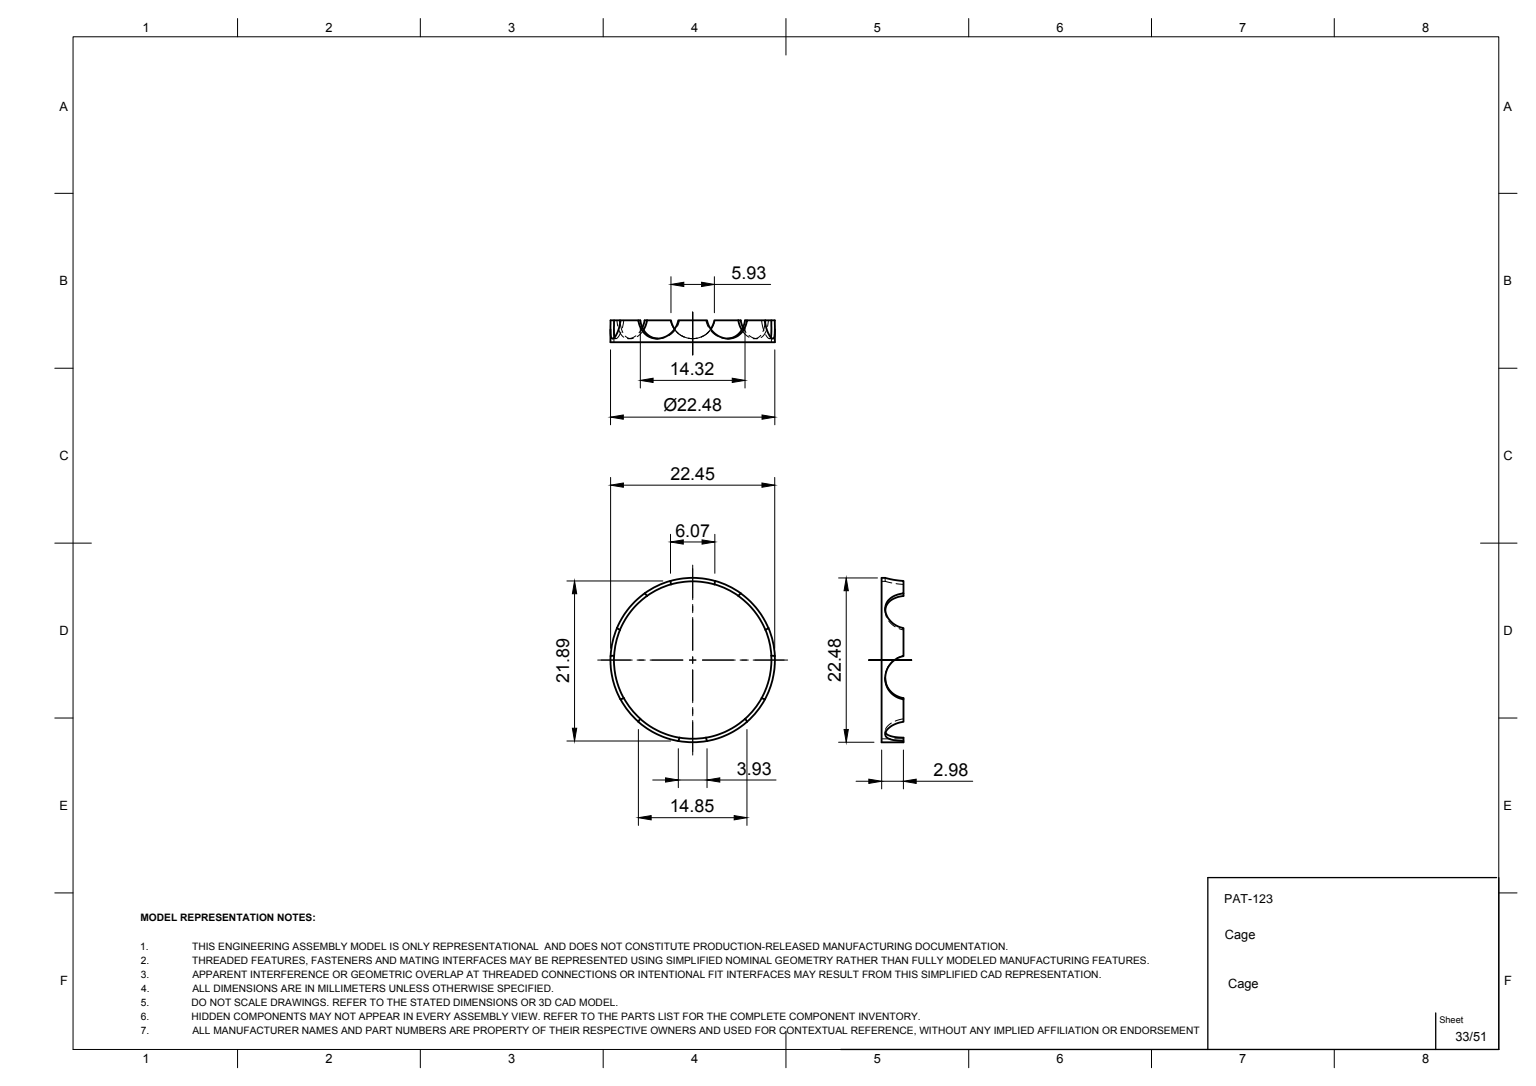
ISO-10303-21;
HEADER;
/* Generated by software containing ST-Developer
 * from STEP Tools, Inc. (www.steptools.com) 
 */

FILE_DESCRIPTION(
/* description */ ('Worm-less right-angle friction wheel drive'),
/* implementation_level */ '2;1');

FILE_NAME(
/* name */ 'Cage.step',
/* time_stamp */ '2026-10-28T03:22:36-07:00',
/* author */ (''),
/* organization */ (''),
/* preprocessor_version */ 'ST-DEVELOPER v20.2',
/* originating_system */ 'Autodesk Translation Framework v15.17.0.0',
/* authorisation */ '');

FILE_SCHEMA (('AUTOMOTIVE_DESIGN { 1 0 10303 214 3 1 1 }'));
ENDSEC;

DATA;
#10=MECHANICAL_DESIGN_GEOMETRIC_PRESENTATION_REPRESENTATION('',(#644),#17046);
#442=SPHERICAL_SURFACE('',#9318,0.309556);
#443=SPHERICAL_SURFACE('',#9334,0.309556);
#444=SPHERICAL_SURFACE('',#9339,0.309556);
#445=SPHERICAL_SURFACE('',#9345,0.309556);
#446=SPHERICAL_SURFACE('',#9350,0.309556);
#447=SPHERICAL_SURFACE('',#9355,0.309556);
#448=SPHERICAL_SURFACE('',#9363,0.309556);
#483=B_SPLINE_CURVE_WITH_KNOTS('',3,(#15498,#15499,#15500,#15501,#15502,
#15503,#15504,#15505,#15506,#15507,#15508,#15509,#15510,#15511,#15512,#15513,
#15514,#15515,#15516,#15517,#15518,#15519),.UNSPECIFIED.,.F.,.F.,(4,2,2,
2,2,2,2,2,2,2,4),(0.0591825211272536,0.157966726598481,0.236950089897721,
0.315933453196962,0.391576304923761,0.46721915665056,0.54286200837736,0.618504860104159,
0.697488223403399,0.77647158670264,0.875255792173867),.UNSPECIFIED.);
#484=B_SPLINE_CURVE_WITH_KNOTS('',3,(#15523,#15524,#15525,#15526,#15527,
#15528,#15529,#15530,#15531,#15532,#15533,#15534,#15535,#15536,#15537,#15538,
#15539,#15540,#15541,#15542,#15543,#15544),.UNSPECIFIED.,.F.,.F.,(4,2,2,
2,2,2,2,2,2,2,4),(0.0581119756758434,0.106553146291161,0.213106292582322,
0.30849933801665,0.386091982889075,0.4636846277615,0.541277272633925,0.61886991750635,
0.714262962940678,0.820816109231839,0.869257279847157),.UNSPECIFIED.);
#485=B_SPLINE_CURVE_WITH_KNOTS('',3,(#15550,#15551,#15552,#15553,#15554,
#15555,#15556,#15557,#15558,#15559,#15560,#15561,#15562,#15563,#15564,#15565,
#15566,#15567,#15568,#15569,#15570,#15571),.UNSPECIFIED.,.F.,.F.,(4,2,2,
2,2,2,2,2,2,2,4),(0.0581119756758434,0.106553146291161,0.213106292582322,
0.30849933801665,0.386091982889075,0.4636846277615,0.541277272633925,0.61886991750635,
0.714262962940679,0.820816109231839,0.869257279847157),.UNSPECIFIED.);
#486=B_SPLINE_CURVE_WITH_KNOTS('',3,(#15575,#15576,#15577,#15578,#15579,
#15580,#15581,#15582,#15583,#15584,#15585,#15586,#15587,#15588,#15589,#15590,
#15591,#15592,#15593,#15594,#15595,#15596),.UNSPECIFIED.,.F.,.F.,(4,2,2,
2,2,2,2,2,2,2,4),(0.0581119756758433,0.106553146291161,0.213106292582322,
0.308499338016649,0.386091982889075,0.4636846277615,0.541277272633925,0.61886991750635,
0.714262962940678,0.820816109231839,0.869257279847157),.UNSPECIFIED.);
#487=B_SPLINE_CURVE_WITH_KNOTS('',3,(#15605,#15606,#15607,#15608,#15609,
#15610,#15611,#15612,#15613,#15614,#15615,#15616,#15617,#15618,#15619,#15620,
#15621,#15622,#15623,#15624,#15625,#15626),.UNSPECIFIED.,.F.,.F.,(4,2,2,
2,2,2,2,2,2,2,4),(0.0581119756758433,0.106553146291161,0.213106292582322,
0.30849933801665,0.386091982889075,0.4636846277615,0.541277272633925,0.61886991750635,
0.714262962940678,0.820816109231839,0.869257279847157),.UNSPECIFIED.);
#488=B_SPLINE_CURVE_WITH_KNOTS('',3,(#15630,#15631,#15632,#15633,#15634,
#15635,#15636,#15637,#15638,#15639,#15640,#15641,#15642,#15643,#15644,#15645,
#15646,#15647,#15648,#15649,#15650,#15651),.UNSPECIFIED.,.F.,.F.,(4,2,2,
2,2,2,2,2,2,2,4),(0.0581119756758434,0.106553146291161,0.213106292582322,
0.30849933801665,0.386091982889075,0.4636846277615,0.541277272633925,0.61886991750635,
0.714262962940678,0.820816109231839,0.869257279847157),.UNSPECIFIED.);
#489=B_SPLINE_CURVE_WITH_KNOTS('',3,(#15655,#15656,#15657,#15658,#15659,
#15660,#15661,#15662,#15663,#15664,#15665,#15666,#15667,#15668,#15669,#15670,
#15671,#15672,#15673,#15674,#15675,#15676),.UNSPECIFIED.,.F.,.F.,(4,2,2,
2,2,2,2,2,2,2,4),(0.0581119756758434,0.106553146291161,0.213106292582322,
0.30849933801665,0.386091982889075,0.4636846277615,0.541277272633925,0.61886991750635,
0.714262962940678,0.820816109231839,0.869257279847157),.UNSPECIFIED.);
#490=B_SPLINE_CURVE_WITH_KNOTS('',3,(#15680,#15681,#15682,#15683,#15684,
#15685,#15686,#15687,#15688,#15689,#15690,#15691,#15692,#15693,#15694,#15695,
#15696,#15697,#15698,#15699,#15700,#15701),.UNSPECIFIED.,.F.,.F.,(4,2,2,
2,2,2,2,2,2,2,4),(0.0581119756758433,0.106553146291161,0.213106292582322,
0.30849933801665,0.386091982889075,0.4636846277615,0.541277272633925,0.61886991750635,
0.714262962940678,0.820816109231839,0.869257279847157),.UNSPECIFIED.);
#491=B_SPLINE_CURVE_WITH_KNOTS('',3,(#15709,#15710,#15711,#15712,#15713,
#15714,#15715,#15716,#15717,#15718,#15719,#15720,#15721,#15722,#15723,#15724,
#15725,#15726,#15727,#15728,#15729,#15730),.UNSPECIFIED.,.F.,.F.,(4,2,2,
2,2,2,2,2,2,2,4),(0.0591825211272536,0.157966726598481,0.236950089897721,
0.315933453196962,0.391576304923761,0.467219156650561,0.54286200837736,
0.618504860104159,0.697488223403399,0.77647158670264,0.875255792173867),
 .UNSPECIFIED.);
#492=B_SPLINE_CURVE_WITH_KNOTS('',3,(#15738,#15739,#15740,#15741,#15742,
#15743,#15744,#15745,#15746,#15747,#15748,#15749,#15750,#15751,#15752,#15753,
#15754,#15755,#15756,#15757,#15758,#15759),.UNSPECIFIED.,.F.,.F.,(4,2,2,
2,2,2,2,2,2,2,4),(0.0591825211272536,0.157966726598481,0.236950089897722,
0.315933453196962,0.391576304923761,0.467219156650561,0.54286200837736,
0.618504860104159,0.697488223403399,0.77647158670264,0.875255792173867),
 .UNSPECIFIED.);
#493=B_SPLINE_CURVE_WITH_KNOTS('',3,(#15769,#15770,#15771,#15772,#15773,
#15774,#15775,#15776,#15777,#15778,#15779,#15780,#15781,#15782,#15783,#15784,
#15785,#15786,#15787,#15788,#15789,#15790),.UNSPECIFIED.,.F.,.F.,(4,2,2,
2,2,2,2,2,2,2,4),(0.0591825211272536,0.157966726598481,0.236950089897721,
0.315933453196962,0.391576304923761,0.46721915665056,0.54286200837736,0.618504860104159,
0.697488223403399,0.77647158670264,0.875255792173867),.UNSPECIFIED.);
#494=B_SPLINE_CURVE_WITH_KNOTS('',3,(#15798,#15799,#15800,#15801,#15802,
#15803,#15804,#15805,#15806,#15807,#15808,#15809,#15810,#15811,#15812,#15813,
#15814,#15815,#15816,#15817,#15818,#15819),.UNSPECIFIED.,.F.,.F.,(4,2,2,
2,2,2,2,2,2,2,4),(0.0591825211272536,0.157966726598481,0.236950089897721,
0.315933453196962,0.391576304923761,0.46721915665056,0.542862008377359,
0.618504860104159,0.697488223403399,0.776471586702639,0.875255792173867),
 .UNSPECIFIED.);
#495=B_SPLINE_CURVE_WITH_KNOTS('',3,(#15827,#15828,#15829,#15830,#15831,
#15832,#15833,#15834,#15835,#15836,#15837,#15838,#15839,#15840,#15841,#15842,
#15843,#15844,#15845,#15846,#15847,#15848),.UNSPECIFIED.,.F.,.F.,(4,2,2,
2,2,2,2,2,2,2,4),(0.0591825211272536,0.157966726598481,0.236950089897721,
0.315933453196962,0.391576304923761,0.46721915665056,0.54286200837736,0.618504860104159,
0.697488223403399,0.77647158670264,0.875255792173867),.UNSPECIFIED.);
#496=B_SPLINE_CURVE_WITH_KNOTS('',3,(#15857,#15858,#15859,#15860,#15861,
#15862,#15863,#15864,#15865,#15866,#15867,#15868,#15869,#15870,#15871,#15872,
#15873,#15874,#15875,#15876,#15877,#15878),.UNSPECIFIED.,.F.,.F.,(4,2,2,
2,2,2,2,2,2,2,4),(0.0591825211272536,0.157966726598481,0.236950089897721,
0.315933453196962,0.391576304923761,0.46721915665056,0.542862008377359,
0.618504860104159,0.697488223403399,0.776471586702639,0.875255792173867),
 .UNSPECIFIED.);
#544=SHAPE_REPRESENTATION_RELATIONSHIP('SRR','None',#17288,#591);
#591=ADVANCED_BREP_SHAPE_REPRESENTATION('',(#697),#17024);
#644=STYLED_ITEM('',(#17591),#697);
#697=MANIFOLD_SOLID_BREP('Continuous crown cage',#8200);
#910=FACE_BOUND('',#2159,.T.);
#1083=PLANE('',#9331);
#1084=PLANE('',#9336);
#1085=PLANE('',#9341);
#1086=PLANE('',#9347);
#1087=PLANE('',#9352);
#1088=PLANE('',#9361);
#1089=PLANE('',#9365);
#1090=PLANE('',#9366);
#1482=FACE_OUTER_BOUND('',#2143,.T.);
#1483=FACE_OUTER_BOUND('',#2144,.T.);
#1484=FACE_OUTER_BOUND('',#2145,.T.);
#1485=FACE_OUTER_BOUND('',#2146,.T.);
#1486=FACE_OUTER_BOUND('',#2147,.T.);
#1487=FACE_OUTER_BOUND('',#2148,.T.);
#1488=FACE_OUTER_BOUND('',#2149,.T.);
#1489=FACE_OUTER_BOUND('',#2150,.T.);
#1490=FACE_OUTER_BOUND('',#2151,.T.);
#1491=FACE_OUTER_BOUND('',#2152,.T.);
#1492=FACE_OUTER_BOUND('',#2153,.T.);
#1493=FACE_OUTER_BOUND('',#2154,.T.);
#1494=FACE_OUTER_BOUND('',#2155,.T.);
#1495=FACE_OUTER_BOUND('',#2156,.T.);
#1496=FACE_OUTER_BOUND('',#2157,.T.);
#1497=FACE_OUTER_BOUND('',#2158,.T.);
#1498=FACE_OUTER_BOUND('',#2160,.T.);
#2143=EDGE_LOOP('',(#6744,#6745,#6746,#6747));
#2144=EDGE_LOOP('',(#6748,#6749,#6750,#6751,#6752,#6753,#6754,#6755,#6756,
#6757,#6758,#6759,#6760,#6761,#6762,#6763,#6764,#6765));
#2145=EDGE_LOOP('',(#6766,#6767,#6768,#6769));
#2146=EDGE_LOOP('',(#6770,#6771,#6772,#6773));
#2147=EDGE_LOOP('',(#6774,#6775,#6776,#6777));
#2148=EDGE_LOOP('',(#6778,#6779,#6780,#6781));
#2149=EDGE_LOOP('',(#6782,#6783,#6784,#6785,#6786,#6787));
#2150=EDGE_LOOP('',(#6788,#6789,#6790,#6791));
#2151=EDGE_LOOP('',(#6792,#6793,#6794,#6795));
#2152=EDGE_LOOP('',(#6796,#6797,#6798,#6799));
#2153=EDGE_LOOP('',(#6800,#6801,#6802,#6803));
#2154=EDGE_LOOP('',(#6804,#6805,#6806,#6807));
#2155=EDGE_LOOP('',(#6808,#6809,#6810,#6811,#6812,#6813,#6814,#6815,#6816,
#6817,#6818,#6819,#6820,#6821,#6822,#6823,#6824,#6825));
#2156=EDGE_LOOP('',(#6826,#6827,#6828,#6829));
#2157=EDGE_LOOP('',(#6830,#6831,#6832,#6833));
#2158=EDGE_LOOP('',(#6834));
#2159=EDGE_LOOP('',(#6835));
#2160=EDGE_LOOP('',(#6836,#6837,#6838,#6839));
#2707=LINE('',#15600,#3247);
#2708=LINE('',#15853,#3248);
#3247=VECTOR('',#11269,1.123812);
#3248=VECTOR('',#11338,1.076188);
#3730=CIRCLE('',#9319,0.303778037777585);
#3731=CIRCLE('',#9320,0.303778037777585);
#3732=CIRCLE('',#9322,1.123812);
#3733=CIRCLE('',#9323,1.123812);
#3734=CIRCLE('',#9324,1.123812);
#3735=CIRCLE('',#9325,1.123812);
#3736=CIRCLE('',#9326,1.123812);
#3737=CIRCLE('',#9327,1.123812);
#3738=CIRCLE('',#9328,1.123812);
#3739=CIRCLE('',#9329,1.123812);
#3740=CIRCLE('',#9330,1.123812);
#3741=CIRCLE('',#9332,1.076188);
#3742=CIRCLE('',#9333,0.303778037777585);
#3743=CIRCLE('',#9335,0.303778037777585);
#3744=CIRCLE('',#9337,1.076188);
#3745=CIRCLE('',#9338,0.303778037777585);
#3746=CIRCLE('',#9340,0.303778037777585);
#3747=CIRCLE('',#9342,1.076188);
#3748=CIRCLE('',#9343,1.076188);
#3749=CIRCLE('',#9344,0.303778037777585);
#3750=CIRCLE('',#9346,0.303778037777585);
#3751=CIRCLE('',#9348,1.076188);
#3752=CIRCLE('',#9349,0.303778037777585);
#3753=CIRCLE('',#9351,0.303778037777585);
#3754=CIRCLE('',#9353,1.076188);
#3755=CIRCLE('',#9354,0.303778037777585);
#3756=CIRCLE('',#9356,0.303778037777585);
#3757=CIRCLE('',#9358,1.076188);
#3758=CIRCLE('',#9359,1.076188);
#3759=CIRCLE('',#9360,1.076188);
#3760=CIRCLE('',#9362,0.303778037777585);
#3761=CIRCLE('',#9364,0.303778037777585);
#4279=VERTEX_POINT('',#15496);
#4280=VERTEX_POINT('',#15497);
#4281=VERTEX_POINT('',#15520);
#4282=VERTEX_POINT('',#15522);
#4283=VERTEX_POINT('',#15547);
#4284=VERTEX_POINT('',#15549);
#4285=VERTEX_POINT('',#15572);
#4286=VERTEX_POINT('',#15574);
#4287=VERTEX_POINT('',#15597);
#4288=VERTEX_POINT('',#15599);
#4289=VERTEX_POINT('',#15602);
#4290=VERTEX_POINT('',#15604);
#4291=VERTEX_POINT('',#15627);
#4292=VERTEX_POINT('',#15629);
#4293=VERTEX_POINT('',#15652);
#4294=VERTEX_POINT('',#15654);
#4295=VERTEX_POINT('',#15677);
#4296=VERTEX_POINT('',#15679);
#4297=VERTEX_POINT('',#15704);
#4298=VERTEX_POINT('',#15708);
#4299=VERTEX_POINT('',#15733);
#4300=VERTEX_POINT('',#15737);
#4301=VERTEX_POINT('',#15762);
#4302=VERTEX_POINT('',#15764);
#4303=VERTEX_POINT('',#15768);
#4304=VERTEX_POINT('',#15793);
#4305=VERTEX_POINT('',#15797);
#4306=VERTEX_POINT('',#15822);
#4307=VERTEX_POINT('',#15826);
#4308=VERTEX_POINT('',#15851);
#4309=VERTEX_POINT('',#15854);
#4310=VERTEX_POINT('',#15856);
#5141=EDGE_CURVE('',#4279,#4280,#483,.T.);
#5142=EDGE_CURVE('',#4281,#4279,#3730,.T.);
#5143=EDGE_CURVE('',#4282,#4281,#484,.T.);
#5144=EDGE_CURVE('',#4280,#4282,#3731,.T.);
#5145=EDGE_CURVE('',#4283,#4281,#3732,.T.);
#5146=EDGE_CURVE('',#4283,#4284,#485,.T.);
#5147=EDGE_CURVE('',#4285,#4284,#3733,.T.);
#5148=EDGE_CURVE('',#4285,#4286,#486,.T.);
#5149=EDGE_CURVE('',#4287,#4286,#3734,.T.);
#5150=EDGE_CURVE('',#4287,#4288,#2707,.T.);
#5151=EDGE_CURVE('',#4288,#4288,#3735,.T.);
#5152=EDGE_CURVE('',#4289,#4287,#3736,.T.);
#5153=EDGE_CURVE('',#4289,#4290,#487,.T.);
#5154=EDGE_CURVE('',#4291,#4290,#3737,.T.);
#5155=EDGE_CURVE('',#4291,#4292,#488,.T.);
#5156=EDGE_CURVE('',#4293,#4292,#3738,.T.);
#5157=EDGE_CURVE('',#4293,#4294,#489,.T.);
#5158=EDGE_CURVE('',#4295,#4294,#3739,.T.);
#5159=EDGE_CURVE('',#4295,#4296,#490,.T.);
#5160=EDGE_CURVE('',#4282,#4296,#3740,.T.);
#5161=EDGE_CURVE('',#4279,#4297,#3741,.T.);
#5162=EDGE_CURVE('',#4297,#4283,#3742,.T.);
#5163=EDGE_CURVE('',#4298,#4297,#491,.T.);
#5164=EDGE_CURVE('',#4284,#4298,#3743,.T.);
#5165=EDGE_CURVE('',#4298,#4299,#3744,.T.);
#5166=EDGE_CURVE('',#4299,#4285,#3745,.T.);
#5167=EDGE_CURVE('',#4300,#4299,#492,.T.);
#5168=EDGE_CURVE('',#4286,#4300,#3746,.T.);
#5169=EDGE_CURVE('',#4300,#4301,#3747,.T.);
#5170=EDGE_CURVE('',#4301,#4302,#3748,.T.);
#5171=EDGE_CURVE('',#4302,#4289,#3749,.T.);
#5172=EDGE_CURVE('',#4303,#4302,#493,.T.);
#5173=EDGE_CURVE('',#4290,#4303,#3750,.T.);
#5174=EDGE_CURVE('',#4303,#4304,#3751,.T.);
#5175=EDGE_CURVE('',#4304,#4291,#3752,.T.);
#5176=EDGE_CURVE('',#4305,#4304,#494,.T.);
#5177=EDGE_CURVE('',#4292,#4305,#3753,.T.);
#5178=EDGE_CURVE('',#4305,#4306,#3754,.T.);
#5179=EDGE_CURVE('',#4306,#4293,#3755,.T.);
#5180=EDGE_CURVE('',#4307,#4306,#495,.T.);
#5181=EDGE_CURVE('',#4294,#4307,#3756,.T.);
#5182=EDGE_CURVE('',#4308,#4308,#3757,.T.);
#5183=EDGE_CURVE('',#4308,#4301,#2708,.T.);
#5184=EDGE_CURVE('',#4309,#4280,#3758,.T.);
#5185=EDGE_CURVE('',#4309,#4310,#496,.T.);
#5186=EDGE_CURVE('',#4307,#4310,#3759,.T.);
#5187=EDGE_CURVE('',#4296,#4309,#3760,.T.);
#5188=EDGE_CURVE('',#4310,#4295,#3761,.T.);
#6744=ORIENTED_EDGE('',*,*,#5141,.F.);
#6745=ORIENTED_EDGE('',*,*,#5142,.F.);
#6746=ORIENTED_EDGE('',*,*,#5143,.F.);
#6747=ORIENTED_EDGE('',*,*,#5144,.F.);
#6748=ORIENTED_EDGE('',*,*,#5143,.T.);
#6749=ORIENTED_EDGE('',*,*,#5145,.F.);
#6750=ORIENTED_EDGE('',*,*,#5146,.T.);
#6751=ORIENTED_EDGE('',*,*,#5147,.F.);
#6752=ORIENTED_EDGE('',*,*,#5148,.T.);
#6753=ORIENTED_EDGE('',*,*,#5149,.F.);
#6754=ORIENTED_EDGE('',*,*,#5150,.T.);
#6755=ORIENTED_EDGE('',*,*,#5151,.F.);
#6756=ORIENTED_EDGE('',*,*,#5150,.F.);
#6757=ORIENTED_EDGE('',*,*,#5152,.F.);
#6758=ORIENTED_EDGE('',*,*,#5153,.T.);
#6759=ORIENTED_EDGE('',*,*,#5154,.F.);
#6760=ORIENTED_EDGE('',*,*,#5155,.T.);
#6761=ORIENTED_EDGE('',*,*,#5156,.F.);
#6762=ORIENTED_EDGE('',*,*,#5157,.T.);
#6763=ORIENTED_EDGE('',*,*,#5158,.F.);
#6764=ORIENTED_EDGE('',*,*,#5159,.T.);
#6765=ORIENTED_EDGE('',*,*,#5160,.F.);
#6766=ORIENTED_EDGE('',*,*,#5142,.T.);
#6767=ORIENTED_EDGE('',*,*,#5161,.T.);
#6768=ORIENTED_EDGE('',*,*,#5162,.T.);
#6769=ORIENTED_EDGE('',*,*,#5145,.T.);
#6770=ORIENTED_EDGE('',*,*,#5163,.F.);
#6771=ORIENTED_EDGE('',*,*,#5164,.F.);
#6772=ORIENTED_EDGE('',*,*,#5146,.F.);
#6773=ORIENTED_EDGE('',*,*,#5162,.F.);
#6774=ORIENTED_EDGE('',*,*,#5164,.T.);
#6775=ORIENTED_EDGE('',*,*,#5165,.T.);
#6776=ORIENTED_EDGE('',*,*,#5166,.T.);
#6777=ORIENTED_EDGE('',*,*,#5147,.T.);
#6778=ORIENTED_EDGE('',*,*,#5167,.F.);
#6779=ORIENTED_EDGE('',*,*,#5168,.F.);
#6780=ORIENTED_EDGE('',*,*,#5148,.F.);
#6781=ORIENTED_EDGE('',*,*,#5166,.F.);
#6782=ORIENTED_EDGE('',*,*,#5168,.T.);
#6783=ORIENTED_EDGE('',*,*,#5169,.T.);
#6784=ORIENTED_EDGE('',*,*,#5170,.T.);
#6785=ORIENTED_EDGE('',*,*,#5171,.T.);
#6786=ORIENTED_EDGE('',*,*,#5152,.T.);
#6787=ORIENTED_EDGE('',*,*,#5149,.T.);
#6788=ORIENTED_EDGE('',*,*,#5172,.F.);
#6789=ORIENTED_EDGE('',*,*,#5173,.F.);
#6790=ORIENTED_EDGE('',*,*,#5153,.F.);
#6791=ORIENTED_EDGE('',*,*,#5171,.F.);
#6792=ORIENTED_EDGE('',*,*,#5173,.T.);
#6793=ORIENTED_EDGE('',*,*,#5174,.T.);
#6794=ORIENTED_EDGE('',*,*,#5175,.T.);
#6795=ORIENTED_EDGE('',*,*,#5154,.T.);
#6796=ORIENTED_EDGE('',*,*,#5176,.F.);
#6797=ORIENTED_EDGE('',*,*,#5177,.F.);
#6798=ORIENTED_EDGE('',*,*,#5155,.F.);
#6799=ORIENTED_EDGE('',*,*,#5175,.F.);
#6800=ORIENTED_EDGE('',*,*,#5177,.T.);
#6801=ORIENTED_EDGE('',*,*,#5178,.T.);
#6802=ORIENTED_EDGE('',*,*,#5179,.T.);
#6803=ORIENTED_EDGE('',*,*,#5156,.T.);
#6804=ORIENTED_EDGE('',*,*,#5157,.F.);
#6805=ORIENTED_EDGE('',*,*,#5179,.F.);
#6806=ORIENTED_EDGE('',*,*,#5180,.F.);
#6807=ORIENTED_EDGE('',*,*,#5181,.F.);
#6808=ORIENTED_EDGE('',*,*,#5182,.F.);
#6809=ORIENTED_EDGE('',*,*,#5183,.T.);
#6810=ORIENTED_EDGE('',*,*,#5169,.F.);
#6811=ORIENTED_EDGE('',*,*,#5167,.T.);
#6812=ORIENTED_EDGE('',*,*,#5165,.F.);
#6813=ORIENTED_EDGE('',*,*,#5163,.T.);
#6814=ORIENTED_EDGE('',*,*,#5161,.F.);
#6815=ORIENTED_EDGE('',*,*,#5141,.T.);
#6816=ORIENTED_EDGE('',*,*,#5184,.F.);
#6817=ORIENTED_EDGE('',*,*,#5185,.T.);
#6818=ORIENTED_EDGE('',*,*,#5186,.F.);
#6819=ORIENTED_EDGE('',*,*,#5180,.T.);
#6820=ORIENTED_EDGE('',*,*,#5178,.F.);
#6821=ORIENTED_EDGE('',*,*,#5176,.T.);
#6822=ORIENTED_EDGE('',*,*,#5174,.F.);
#6823=ORIENTED_EDGE('',*,*,#5172,.T.);
#6824=ORIENTED_EDGE('',*,*,#5170,.F.);
#6825=ORIENTED_EDGE('',*,*,#5183,.F.);
#6826=ORIENTED_EDGE('',*,*,#5144,.T.);
#6827=ORIENTED_EDGE('',*,*,#5160,.T.);
#6828=ORIENTED_EDGE('',*,*,#5187,.T.);
#6829=ORIENTED_EDGE('',*,*,#5184,.T.);
#6830=ORIENTED_EDGE('',*,*,#5159,.F.);
#6831=ORIENTED_EDGE('',*,*,#5188,.F.);
#6832=ORIENTED_EDGE('',*,*,#5185,.F.);
#6833=ORIENTED_EDGE('',*,*,#5187,.F.);
#6834=ORIENTED_EDGE('',*,*,#5151,.T.);
#6835=ORIENTED_EDGE('',*,*,#5182,.T.);
#6836=ORIENTED_EDGE('',*,*,#5181,.T.);
#6837=ORIENTED_EDGE('',*,*,#5186,.T.);
#6838=ORIENTED_EDGE('',*,*,#5188,.T.);
#6839=ORIENTED_EDGE('',*,*,#5158,.T.);
#7654=CYLINDRICAL_SURFACE('',#9321,1.123812);
#7655=CYLINDRICAL_SURFACE('',#9357,1.076188);
#7974=ADVANCED_FACE('',(#1482),#442,.F.);
#7975=ADVANCED_FACE('',(#1483),#7654,.T.);
#7976=ADVANCED_FACE('',(#1484),#1083,.T.);
#7977=ADVANCED_FACE('',(#1485),#443,.F.);
#7978=ADVANCED_FACE('',(#1486),#1084,.T.);
#7979=ADVANCED_FACE('',(#1487),#444,.F.);
#7980=ADVANCED_FACE('',(#1488),#1085,.T.);
#7981=ADVANCED_FACE('',(#1489),#445,.F.);
#7982=ADVANCED_FACE('',(#1490),#1086,.T.);
#7983=ADVANCED_FACE('',(#1491),#446,.F.);
#7984=ADVANCED_FACE('',(#1492),#1087,.T.);
#7985=ADVANCED_FACE('',(#1493),#447,.F.);
#7986=ADVANCED_FACE('',(#1494),#7655,.F.);
#7987=ADVANCED_FACE('',(#1495),#1088,.T.);
#7988=ADVANCED_FACE('',(#1496),#448,.F.);
#7989=ADVANCED_FACE('',(#1497,#910),#1089,.T.);
#7990=ADVANCED_FACE('',(#1498),#1090,.T.);
#8200=CLOSED_SHELL('',(#7974,#7975,#7976,#7977,#7978,#7979,#7980,#7981,
#7982,#7983,#7984,#7985,#7986,#7987,#7988,#7989,#7990));
#9317=AXIS2_PLACEMENT_3D('',#15494,#11253,#11254);
#9318=AXIS2_PLACEMENT_3D('',#15495,#11255,#11256);
#9319=AXIS2_PLACEMENT_3D('',#15521,#11257,#11258);
#9320=AXIS2_PLACEMENT_3D('',#15545,#11259,#11260);
#9321=AXIS2_PLACEMENT_3D('',#15546,#11261,#11262);
#9322=AXIS2_PLACEMENT_3D('',#15548,#11263,#11264);
#9323=AXIS2_PLACEMENT_3D('',#15573,#11265,#11266);
#9324=AXIS2_PLACEMENT_3D('',#15598,#11267,#11268);
#9325=AXIS2_PLACEMENT_3D('',#15601,#11270,#11271);
#9326=AXIS2_PLACEMENT_3D('',#15603,#11272,#11273);
#9327=AXIS2_PLACEMENT_3D('',#15628,#11274,#11275);
#9328=AXIS2_PLACEMENT_3D('',#15653,#11276,#11277);
#9329=AXIS2_PLACEMENT_3D('',#15678,#11278,#11279);
#9330=AXIS2_PLACEMENT_3D('',#15702,#11280,#11281);
#9331=AXIS2_PLACEMENT_3D('',#15703,#11282,#11283);
#9332=AXIS2_PLACEMENT_3D('',#15705,#11284,#11285);
#9333=AXIS2_PLACEMENT_3D('',#15706,#11286,#11287);
#9334=AXIS2_PLACEMENT_3D('',#15707,#11288,#11289);
#9335=AXIS2_PLACEMENT_3D('',#15731,#11290,#11291);
#9336=AXIS2_PLACEMENT_3D('',#15732,#11292,#11293);
#9337=AXIS2_PLACEMENT_3D('',#15734,#11294,#11295);
#9338=AXIS2_PLACEMENT_3D('',#15735,#11296,#11297);
#9339=AXIS2_PLACEMENT_3D('',#15736,#11298,#11299);
#9340=AXIS2_PLACEMENT_3D('',#15760,#11300,#11301);
#9341=AXIS2_PLACEMENT_3D('',#15761,#11302,#11303);
#9342=AXIS2_PLACEMENT_3D('',#15763,#11304,#11305);
#9343=AXIS2_PLACEMENT_3D('',#15765,#11306,#11307);
#9344=AXIS2_PLACEMENT_3D('',#15766,#11308,#11309);
#9345=AXIS2_PLACEMENT_3D('',#15767,#11310,#11311);
#9346=AXIS2_PLACEMENT_3D('',#15791,#11312,#11313);
#9347=AXIS2_PLACEMENT_3D('',#15792,#11314,#11315);
#9348=AXIS2_PLACEMENT_3D('',#15794,#11316,#11317);
#9349=AXIS2_PLACEMENT_3D('',#15795,#11318,#11319);
#9350=AXIS2_PLACEMENT_3D('',#15796,#11320,#11321);
#9351=AXIS2_PLACEMENT_3D('',#15820,#11322,#11323);
#9352=AXIS2_PLACEMENT_3D('',#15821,#11324,#11325);
#9353=AXIS2_PLACEMENT_3D('',#15823,#11326,#11327);
#9354=AXIS2_PLACEMENT_3D('',#15824,#11328,#11329);
#9355=AXIS2_PLACEMENT_3D('',#15825,#11330,#11331);
#9356=AXIS2_PLACEMENT_3D('',#15849,#11332,#11333);
#9357=AXIS2_PLACEMENT_3D('',#15850,#11334,#11335);
#9358=AXIS2_PLACEMENT_3D('',#15852,#11336,#11337);
#9359=AXIS2_PLACEMENT_3D('',#15855,#11339,#11340);
#9360=AXIS2_PLACEMENT_3D('',#15879,#11341,#11342);
#9361=AXIS2_PLACEMENT_3D('',#15880,#11343,#11344);
#9362=AXIS2_PLACEMENT_3D('',#15881,#11345,#11346);
#9363=AXIS2_PLACEMENT_3D('',#15882,#11347,#11348);
#9364=AXIS2_PLACEMENT_3D('',#15883,#11349,#11350);
#9365=AXIS2_PLACEMENT_3D('',#15884,#11351,#11352);
#9366=AXIS2_PLACEMENT_3D('',#15885,#11353,#11354);
#11253=DIRECTION('axis',(0.,0.,1.));
#11254=DIRECTION('refdir',(1.,0.,0.));
#11255=DIRECTION('center_axis',(0.,0.,1.));
#11256=DIRECTION('ref_axis',(1.,0.,0.));
#11257=DIRECTION('center_axis',(0.,-1.,0.));
#11258=DIRECTION('ref_axis',(0.,0.,-1.));
#11259=DIRECTION('center_axis',(0.,-1.,0.));
#11260=DIRECTION('ref_axis',(0.,0.,-1.));
#11261=DIRECTION('center_axis',(0.,1.,0.));
#11262=DIRECTION('ref_axis',(1.,0.,0.));
#11263=DIRECTION('center_axis',(0.,1.,0.));
#11264=DIRECTION('ref_axis',(1.,0.,0.));
#11265=DIRECTION('center_axis',(0.,1.,0.));
#11266=DIRECTION('ref_axis',(1.,0.,0.));
#11267=DIRECTION('center_axis',(0.,1.,0.));
#11268=DIRECTION('ref_axis',(1.,0.,0.));
#11269=DIRECTION('',(0.,-1.,0.));
#11270=DIRECTION('center_axis',(0.,-1.,0.));
#11271=DIRECTION('ref_axis',(1.,0.,0.));
#11272=DIRECTION('center_axis',(0.,1.,0.));
#11273=DIRECTION('ref_axis',(1.,0.,0.));
#11274=DIRECTION('center_axis',(0.,1.,0.));
#11275=DIRECTION('ref_axis',(1.,0.,0.));
#11276=DIRECTION('center_axis',(0.,1.,0.));
#11277=DIRECTION('ref_axis',(1.,0.,0.));
#11278=DIRECTION('center_axis',(0.,1.,0.));
#11279=DIRECTION('ref_axis',(1.,0.,0.));
#11280=DIRECTION('center_axis',(0.,1.,0.));
#11281=DIRECTION('ref_axis',(1.,0.,0.));
#11282=DIRECTION('center_axis',(0.,1.,0.));
#11283=DIRECTION('ref_axis',(1.,0.,0.));
#11284=DIRECTION('center_axis',(0.,-1.,0.));
#11285=DIRECTION('ref_axis',(1.,0.,0.));
#11286=DIRECTION('center_axis',(0.,-1.,0.));
#11287=DIRECTION('ref_axis',(0.,0.,-1.));
#11288=DIRECTION('center_axis',(8.96625347776458E-17,0.,1.));
#11289=DIRECTION('ref_axis',(1.,0.,0.));
#11290=DIRECTION('center_axis',(0.,-1.,0.));
#11291=DIRECTION('ref_axis',(0.,0.,-1.));
#11292=DIRECTION('center_axis',(0.,1.,0.));
#11293=DIRECTION('ref_axis',(1.,0.,0.));
#11294=DIRECTION('center_axis',(0.,-1.,0.));
#11295=DIRECTION('ref_axis',(1.,0.,0.));
#11296=DIRECTION('center_axis',(0.,-1.,0.));
#11297=DIRECTION('ref_axis',(0.,0.,-1.));
#11298=DIRECTION('center_axis',(0.,0.,1.));
#11299=DIRECTION('ref_axis',(1.,0.,0.));
#11300=DIRECTION('center_axis',(0.,-1.,0.));
#11301=DIRECTION('ref_axis',(0.,0.,-1.));
#11302=DIRECTION('center_axis',(0.,1.,0.));
#11303=DIRECTION('ref_axis',(1.,0.,0.));
#11304=DIRECTION('center_axis',(0.,-1.,0.));
#11305=DIRECTION('ref_axis',(1.,0.,0.));
#11306=DIRECTION('center_axis',(0.,-1.,0.));
#11307=DIRECTION('ref_axis',(1.,0.,0.));
#11308=DIRECTION('center_axis',(0.,-1.,0.));
#11309=DIRECTION('ref_axis',(0.,0.,-1.));
#11310=DIRECTION('center_axis',(0.,0.,1.));
#11311=DIRECTION('ref_axis',(1.,0.,0.));
#11312=DIRECTION('center_axis',(0.,-1.,0.));
#11313=DIRECTION('ref_axis',(0.,0.,-1.));
#11314=DIRECTION('center_axis',(0.,1.,0.));
#11315=DIRECTION('ref_axis',(1.,0.,0.));
#11316=DIRECTION('center_axis',(0.,-1.,0.));
#11317=DIRECTION('ref_axis',(1.,0.,0.));
#11318=DIRECTION('center_axis',(0.,-1.,0.));
#11319=DIRECTION('ref_axis',(0.,0.,-1.));
#11320=DIRECTION('center_axis',(8.96625347776458E-17,0.,1.));
#11321=DIRECTION('ref_axis',(1.,0.,0.));
#11322=DIRECTION('center_axis',(0.,-1.,0.));
#11323=DIRECTION('ref_axis',(0.,0.,-1.));
#11324=DIRECTION('center_axis',(0.,1.,0.));
#11325=DIRECTION('ref_axis',(1.,0.,0.));
#11326=DIRECTION('center_axis',(0.,-1.,0.));
#11327=DIRECTION('ref_axis',(1.,0.,0.));
#11328=DIRECTION('center_axis',(0.,-1.,0.));
#11329=DIRECTION('ref_axis',(0.,0.,-1.));
#11330=DIRECTION('center_axis',(0.,0.,1.));
#11331=DIRECTION('ref_axis',(1.,0.,0.));
#11332=DIRECTION('center_axis',(0.,-1.,0.));
#11333=DIRECTION('ref_axis',(0.,0.,-1.));
#11334=DIRECTION('center_axis',(0.,1.,0.));
#11335=DIRECTION('ref_axis',(1.,0.,0.));
#11336=DIRECTION('center_axis',(0.,1.,0.));
#11337=DIRECTION('ref_axis',(1.,0.,0.));
#11338=DIRECTION('',(0.,1.,0.));
#11339=DIRECTION('center_axis',(0.,-1.,0.));
#11340=DIRECTION('ref_axis',(1.,0.,0.));
#11341=DIRECTION('center_axis',(0.,-1.,0.));
#11342=DIRECTION('ref_axis',(1.,0.,0.));
#11343=DIRECTION('center_axis',(0.,1.,0.));
#11344=DIRECTION('ref_axis',(1.,0.,0.));
#11345=DIRECTION('center_axis',(0.,-1.,0.));
#11346=DIRECTION('ref_axis',(0.,0.,-1.));
#11347=DIRECTION('center_axis',(0.,0.,1.));
#11348=DIRECTION('ref_axis',(1.,0.,0.));
#11349=DIRECTION('center_axis',(0.,-1.,0.));
#11350=DIRECTION('ref_axis',(0.,0.,-1.));
#11351=DIRECTION('center_axis',(0.,-1.,0.));
#11352=DIRECTION('ref_axis',(-1.,0.,0.));
#11353=DIRECTION('center_axis',(0.,1.,0.));
#11354=DIRECTION('ref_axis',(1.,0.,0.));
#15494=CARTESIAN_POINT('',(0.,0.,0.));
#15495=CARTESIAN_POINT('Origin',(0.685838782044607,0.,0.860014630714833));
#15496=CARTESIAN_POINT('',(0.413083465285518,-0.05953,0.993751811093549));
#15497=CARTESIAN_POINT('',(0.876916659919095,-0.05953,0.623857181492959));
#15498=CARTESIAN_POINT('Ctrl Pts',(0.413083465285518,-0.05953,0.993751811093549));
#15499=CARTESIAN_POINT('Ctrl Pts',(0.419070565453383,-0.0925528133349865,
0.991263089003441));
#15500=CARTESIAN_POINT('Ctrl Pts',(0.430199341854858,-0.124911173756694,
0.986608710139579));
#15501=CARTESIAN_POINT('Ctrl Pts',(0.457978755888596,-0.177924977804098,
0.973971221090534));
#15502=CARTESIAN_POINT('Ctrl Pts',(0.473077587363685,-0.199697230012983,
0.966820759530997));
#15503=CARTESIAN_POINT('Ctrl Pts',(0.507057380724533,-0.237895043532788,
0.949440676105255));
#15504=CARTESIAN_POINT('Ctrl Pts',(0.525933334162555,-0.254319232363049,
0.939198248544428));
#15505=CARTESIAN_POINT('Ctrl Pts',(0.564362943424238,-0.28018331644634,
0.916597376014514));
#15506=CARTESIAN_POINT('Ctrl Pts',(0.585840553788742,-0.29104845371857,
0.903141581680914));
#15507=CARTESIAN_POINT('Ctrl Pts',(0.629305439856167,-0.30527573347708,
0.873412008702649));
#15508=CARTESIAN_POINT('Ctrl Pts',(0.651278921914856,-0.308638795020976,
0.857118508332695));
#15509=CARTESIAN_POINT('Ctrl Pts',(0.690705563850638,-0.308638795020976,
0.825676810575914));
#15510=CARTESIAN_POINT('Ctrl Pts',(0.711480111898423,-0.30527573347708,
0.807879894508811));
#15511=CARTESIAN_POINT('Ctrl Pts',(0.750136149454208,-0.29104845371857,
0.772120216227122));
#15512=CARTESIAN_POINT('Ctrl Pts',(0.768033796848072,-0.28018331644634,
0.754175290318038));
#15513=CARTESIAN_POINT('Ctrl Pts',(0.798619410861634,-0.254319232363049,
0.721738358858166));
#15514=CARTESIAN_POINT('Ctrl Pts',(0.812805334167529,-0.237895043532788,
0.705614819529209));
#15515=CARTESIAN_POINT('Ctrl Pts',(0.837310877969633,-0.199697230012983,
0.676354402927683));
#15516=CARTESIAN_POINT('Ctrl Pts',(0.847641868610495,-0.177924977804098,
0.663225258065736));
#15517=CARTESIAN_POINT('Ctrl Pts',(0.866144010579847,-0.124911173756694,
0.638954437806245));
#15518=CARTESIAN_POINT('Ctrl Pts',(0.873158080166742,-0.0925528133349865,
0.62914037979579));
#15519=CARTESIAN_POINT('Ctrl Pts',(0.876916659919095,-0.05953,0.623857181492959));
#15520=CARTESIAN_POINT('',(0.437601487681057,-0.05953,1.03511272300331));
#15521=CARTESIAN_POINT('Origin',(0.685838782044607,-0.05953,0.860014630714833));
#15522=CARTESIAN_POINT('',(0.911784794170997,-0.05953,0.656964154625313));
#15523=CARTESIAN_POINT('Ctrl Pts',(0.911784794170998,-0.0595300000000001,
0.656964154625312));
#15524=CARTESIAN_POINT('Ctrl Pts',(0.909827729890942,-0.0762225747374255,
0.659680317203144));
#15525=CARTESIAN_POINT('Ctrl Pts',(0.907004864562642,-0.0928409665394228,
0.663576540841106));
#15526=CARTESIAN_POINT('Ctrl Pts',(0.895234408667242,-0.144299303100741,
0.679480524217551));
#15527=CARTESIAN_POINT('Ctrl Pts',(0.882797231409153,-0.177024326825049,
0.695831250979106));
#15528=CARTESIAN_POINT('Ctrl Pts',(0.854332839576145,-0.227269801620064,
0.73042219438957));
#15529=CARTESIAN_POINT('Ctrl Pts',(0.834863020612702,-0.251265615809407,
0.752807465209441));
#15530=CARTESIAN_POINT('Ctrl Pts',(0.800439809856111,-0.279889827963178,
0.789147407129766));
#15531=CARTESIAN_POINT('Ctrl Pts',(0.781998747691871,-0.290879136862659,
0.80756613568454));
#15532=CARTESIAN_POINT('Ctrl Pts',(0.742239891936898,-0.305251990234487,
0.844254137480382));
#15533=CARTESIAN_POINT('Ctrl Pts',(0.720906778729541,-0.308638795020976,
0.862505527716294));
#15534=CARTESIAN_POINT('Ctrl Pts',(0.680463863683392,-0.308638795020976,
0.894757676234429));
#15535=CARTESIAN_POINT('Ctrl Pts',(0.657923009631182,-0.305251990234488,
0.91149460735272));
#15536=CARTESIAN_POINT('Ctrl Pts',(0.613307674922609,-0.290879136862659,
0.942092777160053));
#15537=CARTESIAN_POINT('Ctrl Pts',(0.591247219971725,-0.279889827963178,
0.955972930713954));
#15538=CARTESIAN_POINT('Ctrl Pts',(0.548158511259202,-0.251265615809407,
0.981446681891443));
#15539=CARTESIAN_POINT('Ctrl Pts',(0.522002043615455,-0.227269801620063,
0.995447160474328));
#15540=CARTESIAN_POINT('Ctrl Pts',(0.481944444320713,-0.177024326825049,
1.01550068154148));
#15541=CARTESIAN_POINT('Ctrl Pts',(0.463236132117164,-0.14429930310074,
1.0239876538093));
#15542=CARTESIAN_POINT('Ctrl Pts',(0.445111721969657,-0.0928409665394226,
1.03192403056628));
#15543=CARTESIAN_POINT('Ctrl Pts',(0.440685038163619,-0.0762225747374254,
1.03380912944435));
#15544=CARTESIAN_POINT('Ctrl Pts',(0.437601487681056,-0.05953,1.03511272300331));
#15545=CARTESIAN_POINT('Origin',(0.685838782044607,-0.05953,0.860014630714833));
#15546=CARTESIAN_POINT('Origin',(0.,-0.208355,0.));
#15547=CARTESIAN_POINT('',(0.0548532617164168,-0.05953,1.12247250791415));
#15548=CARTESIAN_POINT('Origin',(0.,-0.05953,0.));
#15549=CARTESIAN_POINT('',(-0.536443649899848,-0.05953,0.987512846410683));
#15550=CARTESIAN_POINT('Ctrl Pts',(0.0548532617164173,-0.0595300000000001,
1.12247250791414));
#15551=CARTESIAN_POINT('Ctrl Pts',(0.05150947068137,-0.0762225747374254,
1.12263591311425));
#15552=CARTESIAN_POINT('Ctrl Pts',(0.0467032526342597,-0.0928409665394227,
1.12285816383385));
#15553=CARTESIAN_POINT('Ctrl Pts',(0.0269302585198975,-0.144299303100741,
1.12357162229597));
#15554=CARTESIAN_POINT('Ctrl Pts',(0.006392292392153,-0.177024326825049,
1.12404235695137));
#15555=CARTESIAN_POINT('Ctrl Pts',(-0.0383992541984087,-0.227269801620063,
1.12335509974011));
#15556=CARTESIAN_POINT('Ctrl Pts',(-0.0680399972366993,-0.251265615809407,
1.12208997038458));
#15557=CARTESIAN_POINT('Ctrl Pts',(-0.117914228755037,-0.279889827963178,
1.1178344036749));
#15558=CARTESIAN_POINT('Ctrl Pts',(-0.14381238480104,-0.290879136862659,
1.11490049012186));
#15559=CARTESIAN_POINT('Ctrl Pts',(-0.19728546073067,-0.305251990234488,
1.10669035995599));
#15560=CARTESIAN_POINT('Ctrl Pts',(-0.224855950742601,-0.308638795020976,
1.10139101611326));
#15561=CARTESIAN_POINT('Ctrl Pts',(-0.275287440920027,-0.308638795020976,
1.0898803575765));
#15562=CARTESIAN_POINT('Ctrl Pts',(-0.302426893214945,-0.305251990234488,
1.08269251410343));
#15563=CARTESIAN_POINT('Ctrl Pts',(-0.35416671187353,-0.290879136862659,
1.06688848765783));
#15564=CARTESIAN_POINT('Ctrl Pts',(-0.3787731215897,-0.279889827963178,
1.05829506364875));
#15565=CARTESIAN_POINT('Ctrl Pts',(-0.425554672694338,-0.251265615809407,
1.04048957871266));
#15566=CARTESIAN_POINT('Ctrl Pts',(-0.452808978448581,-0.227269801620063,
1.02876878445619));
#15567=CARTESIAN_POINT('Ctrl Pts',(-0.493462957200432,-0.177024326825049,
1.0099536580922));
#15568=CARTESIAN_POINT('Ctrl Pts',(-0.511762781179148,-0.14429930310074,
1.00061845128527));
#15569=CARTESIAN_POINT('Ctrl Pts',(-0.529268075276157,-0.0928409665394226,
0.991396466802468));
#15570=CARTESIAN_POINT('Ctrl Pts',(-0.533501897135713,-0.0762225747374254,
0.989110885965947));
#15571=CARTESIAN_POINT('Ctrl Pts',(-0.536443649899848,-0.0595300000000001,
0.987512846410683));
#15572=CARTESIAN_POINT('',(-0.843383895613249,-0.05953,0.742736168477219));
#15573=CARTESIAN_POINT('Origin',(0.,-0.05953,0.));
#15574=CARTESIAN_POINT('',(-1.10653577764992,-0.05953,0.196295654879792));
#15575=CARTESIAN_POINT('Ctrl Pts',(-0.843383895613249,-0.0595300000000001,
0.742736168477219));
#15576=CARTESIAN_POINT('Ctrl Pts',(-0.84559647055299,-0.0762225747374255,
0.740223768851062));
#15577=CARTESIAN_POINT('Ctrl Pts',(-0.848766861100456,-0.0928409665394227,
0.736604687327351));
#15578=CARTESIAN_POINT('Ctrl Pts',(-0.861652925570091,-0.144299303100741,
0.721590372101268));
#15579=CARTESIAN_POINT('Ctrl Pts',(-0.87482617317514,-0.177024326825049,
0.705826641853758));
#15580=CARTESIAN_POINT('Ctrl Pts',(-0.902215926359523,-0.227269801620063,
0.670378702718353));
#15581=CARTESIAN_POINT('Ctrl Pts',(-0.919707509403859,-0.251265615809407,
0.646415841396062));
#15582=CARTESIAN_POINT('Ctrl Pts',(-0.947476448101718,-0.279889827963178,
0.604769294586516));
#15583=CARTESIAN_POINT('Ctrl Pts',(-0.961329858300736,-0.290879136862659,
0.582692035672022));
#15584=CARTESIAN_POINT('Ctrl Pts',(-0.988250837578047,-0.305251990234488,
0.535766169015486));
#15585=CARTESIAN_POINT('Ctrl Pts',(-1.00129756308006,-0.308638795020976,
0.510906605094603));
#15586=CARTESIAN_POINT('Ctrl Pts',(-1.02374168767024,-0.308638795020976,
0.46430090015576));
#15587=CARTESIAN_POINT('Ctrl Pts',(-1.03504317708586,-0.305251990234488,
0.438600874831839));
#15588=CARTESIAN_POINT('Ctrl Pts',(-1.05494634094458,-0.290879136862659,
0.388295406390235));
#15589=CARTESIAN_POINT('Ctrl Pts',(-1.06356957703048,-0.279889827963178,
0.363699428370917));
#15590=CARTESIAN_POINT('Ctrl Pts',(-1.0788165083757,-0.251265615809407,
0.316022600643821));
#15591=CARTESIAN_POINT('Ctrl Pts',(-1.08664560412098,-0.227269801620063,
0.287406530683752));
#15592=CARTESIAN_POINT('Ctrl Pts',(-1.09728268713976,-0.177024326825049,
0.243890930799337));
#15593=CARTESIAN_POINT('Ctrl Pts',(-1.10139388218929,-0.144299303100741,
0.22376314604679));
#15594=CARTESIAN_POINT('Ctrl Pts',(-1.10509821673782,-0.0928409665394227,
0.204327142733961));
#15595=CARTESIAN_POINT('Ctrl Pts',(-1.10595102243643,-0.0762225747374254,
0.199591971170104));
#15596=CARTESIAN_POINT('Ctrl Pts',(-1.10653577764992,-0.0595300000000001,
0.196295654879792));
#15597=CARTESIAN_POINT('',(-1.123812,-0.05953,1.37627276864339E-16));
#15598=CARTESIAN_POINT('Origin',(0.,-0.05953,0.));
#15599=CARTESIAN_POINT('',(-1.123812,-0.35718,1.37627276864339E-16));
#15600=CARTESIAN_POINT('',(-1.123812,-0.208355,1.37627276864339E-16));
#15601=CARTESIAN_POINT('Origin',(0.,-0.35718,0.));
#15602=CARTESIAN_POINT('',(-1.10653577764992,-0.05953,-0.196295654879793));
#15603=CARTESIAN_POINT('Origin',(0.,-0.05953,0.));
#15604=CARTESIAN_POINT('',(-0.843383895613249,-0.05953,-0.742736168477219));
#15605=CARTESIAN_POINT('Ctrl Pts',(-1.10653577764992,-0.0595300000000001,
-0.196295654879792));
#15606=CARTESIAN_POINT('Ctrl Pts',(-1.10595102243643,-0.0762225747374255,
-0.199591971170104));
#15607=CARTESIAN_POINT('Ctrl Pts',(-1.10509821673782,-0.0928409665394228,
-0.204327142733962));
#15608=CARTESIAN_POINT('Ctrl Pts',(-1.10139388218929,-0.144299303100741,
-0.22376314604679));
#15609=CARTESIAN_POINT('Ctrl Pts',(-1.09728268713976,-0.177024326825049,
-0.243890930799338));
#15610=CARTESIAN_POINT('Ctrl Pts',(-1.08664560412098,-0.227269801620063,
-0.287406530683753));
#15611=CARTESIAN_POINT('Ctrl Pts',(-1.0788165083757,-0.251265615809407,
-0.316022600643821));
#15612=CARTESIAN_POINT('Ctrl Pts',(-1.06356957703048,-0.279889827963178,
-0.363699428370918));
#15613=CARTESIAN_POINT('Ctrl Pts',(-1.05494634094458,-0.290879136862659,
-0.388295406390235));
#15614=CARTESIAN_POINT('Ctrl Pts',(-1.03504317708586,-0.305251990234488,
-0.438600874831839));
#15615=CARTESIAN_POINT('Ctrl Pts',(-1.02374168767024,-0.308638795020976,
-0.46430090015576));
#15616=CARTESIAN_POINT('Ctrl Pts',(-1.00129756308006,-0.308638795020976,
-0.510906605094603));
#15617=CARTESIAN_POINT('Ctrl Pts',(-0.988250837578047,-0.305251990234488,
-0.535766169015486));
#15618=CARTESIAN_POINT('Ctrl Pts',(-0.961329858300736,-0.290879136862659,
-0.582692035672022));
#15619=CARTESIAN_POINT('Ctrl Pts',(-0.947476448101718,-0.279889827963178,
-0.604769294586516));
#15620=CARTESIAN_POINT('Ctrl Pts',(-0.919707509403859,-0.251265615809407,
-0.646415841396062));
#15621=CARTESIAN_POINT('Ctrl Pts',(-0.902215926359523,-0.227269801620064,
-0.670378702718353));
#15622=CARTESIAN_POINT('Ctrl Pts',(-0.87482617317514,-0.177024326825049,
-0.705826641853758));
#15623=CARTESIAN_POINT('Ctrl Pts',(-0.861652925570091,-0.144299303100741,
-0.721590372101268));
#15624=CARTESIAN_POINT('Ctrl Pts',(-0.848766861100456,-0.0928409665394229,
-0.736604687327351));
#15625=CARTESIAN_POINT('Ctrl Pts',(-0.84559647055299,-0.0762225747374255,
-0.740223768851063));
#15626=CARTESIAN_POINT('Ctrl Pts',(-0.843383895613249,-0.0595300000000001,
-0.742736168477219));
#15627=CARTESIAN_POINT('',(-0.536443649899847,-0.05953,-0.987512846410683));
#15628=CARTESIAN_POINT('Origin',(0.,-0.05953,0.));
#15629=CARTESIAN_POINT('',(0.0548532617164172,-0.05953,-1.12247250791415));
#15630=CARTESIAN_POINT('Ctrl Pts',(-0.536443649899848,-0.0595300000000001,
-0.987512846410683));
#15631=CARTESIAN_POINT('Ctrl Pts',(-0.533501897135712,-0.0762225747374254,
-0.989110885965947));
#15632=CARTESIAN_POINT('Ctrl Pts',(-0.529268075276156,-0.0928409665394227,
-0.991396466802469));
#15633=CARTESIAN_POINT('Ctrl Pts',(-0.511762781179147,-0.144299303100741,
-1.00061845128527));
#15634=CARTESIAN_POINT('Ctrl Pts',(-0.493462957200432,-0.177024326825049,
-1.0099536580922));
#15635=CARTESIAN_POINT('Ctrl Pts',(-0.45280897844858,-0.227269801620063,
-1.02876878445619));
#15636=CARTESIAN_POINT('Ctrl Pts',(-0.425554672694337,-0.251265615809407,
-1.04048957871266));
#15637=CARTESIAN_POINT('Ctrl Pts',(-0.3787731215897,-0.279889827963178,
-1.05829506364875));
#15638=CARTESIAN_POINT('Ctrl Pts',(-0.354166711873529,-0.290879136862659,
-1.06688848765783));
#15639=CARTESIAN_POINT('Ctrl Pts',(-0.302426893214944,-0.305251990234488,
-1.08269251410343));
#15640=CARTESIAN_POINT('Ctrl Pts',(-0.275287440920027,-0.308638795020976,
-1.0898803575765));
#15641=CARTESIAN_POINT('Ctrl Pts',(-0.224855950742601,-0.308638795020976,
-1.10139101611326));
#15642=CARTESIAN_POINT('Ctrl Pts',(-0.19728546073067,-0.305251990234488,
-1.10669035995599));
#15643=CARTESIAN_POINT('Ctrl Pts',(-0.143812384801039,-0.290879136862659,
-1.11490049012186));
#15644=CARTESIAN_POINT('Ctrl Pts',(-0.117914228755037,-0.279889827963178,
-1.1178344036749));
#15645=CARTESIAN_POINT('Ctrl Pts',(-0.0680399972366989,-0.251265615809407,
-1.12208997038458));
#15646=CARTESIAN_POINT('Ctrl Pts',(-0.0383992541984084,-0.227269801620063,
-1.12335509974011));
#15647=CARTESIAN_POINT('Ctrl Pts',(0.00639229239215326,-0.177024326825049,
-1.12404235695137));
#15648=CARTESIAN_POINT('Ctrl Pts',(0.0269302585198977,-0.144299303100741,
-1.12357162229597));
#15649=CARTESIAN_POINT('Ctrl Pts',(0.04670325263426,-0.0928409665394228,
-1.12285816383385));
#15650=CARTESIAN_POINT('Ctrl Pts',(0.0515094706813703,-0.0762225747374255,
-1.12263591311425));
#15651=CARTESIAN_POINT('Ctrl Pts',(0.0548532617164176,-0.0595300000000001,
-1.12247250791414));
#15652=CARTESIAN_POINT('',(0.437601487681057,-0.05953,-1.03511272300331));
#15653=CARTESIAN_POINT('Origin',(0.,-0.05953,0.));
#15654=CARTESIAN_POINT('',(0.911784794170997,-0.05953,-0.656964154625313));
#15655=CARTESIAN_POINT('Ctrl Pts',(0.437601487681056,-0.0595300000000001,
-1.03511272300331));
#15656=CARTESIAN_POINT('Ctrl Pts',(0.440685038163619,-0.0762225747374255,
-1.03380912944435));
#15657=CARTESIAN_POINT('Ctrl Pts',(0.445111721969657,-0.0928409665394228,
-1.03192403056628));
#15658=CARTESIAN_POINT('Ctrl Pts',(0.463236132117164,-0.144299303100741,
-1.0239876538093));
#15659=CARTESIAN_POINT('Ctrl Pts',(0.481944444320713,-0.177024326825049,
-1.01550068154148));
#15660=CARTESIAN_POINT('Ctrl Pts',(0.522002043615455,-0.227269801620064,
-0.995447160474328));
#15661=CARTESIAN_POINT('Ctrl Pts',(0.548158511259203,-0.251265615809407,
-0.981446681891443));
#15662=CARTESIAN_POINT('Ctrl Pts',(0.591247219971725,-0.279889827963178,
-0.955972930713954));
#15663=CARTESIAN_POINT('Ctrl Pts',(0.613307674922609,-0.290879136862659,
-0.942092777160053));
#15664=CARTESIAN_POINT('Ctrl Pts',(0.657923009631182,-0.305251990234487,
-0.91149460735272));
#15665=CARTESIAN_POINT('Ctrl Pts',(0.680463863683393,-0.308638795020976,
-0.894757676234429));
#15666=CARTESIAN_POINT('Ctrl Pts',(0.720906778729542,-0.308638795020976,
-0.862505527716294));
#15667=CARTESIAN_POINT('Ctrl Pts',(0.742239891936899,-0.305251990234488,
-0.844254137480381));
#15668=CARTESIAN_POINT('Ctrl Pts',(0.781998747691872,-0.290879136862659,
-0.80756613568454));
#15669=CARTESIAN_POINT('Ctrl Pts',(0.800439809856112,-0.279889827963178,
-0.789147407129765));
#15670=CARTESIAN_POINT('Ctrl Pts',(0.834863020612702,-0.251265615809407,
-0.752807465209441));
#15671=CARTESIAN_POINT('Ctrl Pts',(0.854332839576145,-0.227269801620064,
-0.73042219438957));
#15672=CARTESIAN_POINT('Ctrl Pts',(0.882797231409153,-0.177024326825049,
-0.695831250979106));
#15673=CARTESIAN_POINT('Ctrl Pts',(0.895234408667242,-0.144299303100741,
-0.679480524217551));
#15674=CARTESIAN_POINT('Ctrl Pts',(0.907004864562642,-0.0928409665394228,
-0.663576540841106));
#15675=CARTESIAN_POINT('Ctrl Pts',(0.909827729890942,-0.0762225747374256,
-0.659680317203144));
#15676=CARTESIAN_POINT('Ctrl Pts',(0.911784794170998,-0.0595300000000001,
-0.656964154625312));
#15677=CARTESIAN_POINT('',(1.08212377959455,-0.05953,-0.303251606722892));
#15678=CARTESIAN_POINT('Origin',(0.,-0.05953,0.));
#15679=CARTESIAN_POINT('',(1.08212377959455,-0.05953,0.303251606722892));
#15680=CARTESIAN_POINT('Ctrl Pts',(1.08212377959455,-0.0595300000000001,
-0.303251606722892));
#15681=CARTESIAN_POINT('Ctrl Pts',(1.0830271513892,-0.0762225747374255,
-0.300028012588062));
#15682=CARTESIAN_POINT('Ctrl Pts',(1.08431331394788,-0.0928409665394228,
-0.2953917518996));
#15683=CARTESIAN_POINT('Ctrl Pts',(1.08940878963422,-0.144299303100741,
-0.276273267473431));
#15684=CARTESIAN_POINT('Ctrl Pts',(1.09443784939331,-0.177024326825049,
-0.256354979351213));
#15685=CARTESIAN_POINT('Ctrl Pts',(1.10373487993589,-0.227269801620064,
-0.212533521233765));
#15686=CARTESIAN_POINT('Ctrl Pts',(1.10909715583869,-0.251265615809407,
-0.183354415742157));
#15687=CARTESIAN_POINT('Ctrl Pts',(1.1160463456491,-0.279889827963178,-0.133783682657561));
#15688=CARTESIAN_POINT('Ctrl Pts',(1.11894887330541,-0.290879136862659,
-0.107881990270302));
#15689=CARTESIAN_POINT('Ctrl Pts',(1.12284346704144,-0.305251990234488,
-0.0539226701638766));
#15690=CARTESIAN_POINT('Ctrl Pts',(1.123812,-0.308638795020976,-0.025864214957475));
#15691=CARTESIAN_POINT('Ctrl Pts',(1.123812,-0.308638795020976,0.025864214957475));
#15692=CARTESIAN_POINT('Ctrl Pts',(1.12284346704144,-0.305251990234488,
0.0539226701638766));
#15693=CARTESIAN_POINT('Ctrl Pts',(1.11894887330541,-0.290879136862659,
0.107881990270302));
#15694=CARTESIAN_POINT('Ctrl Pts',(1.1160463456491,-0.279889827963178,0.133783682657561));
#15695=CARTESIAN_POINT('Ctrl Pts',(1.10909715583869,-0.251265615809407,
0.183354415742157));
#15696=CARTESIAN_POINT('Ctrl Pts',(1.10373487993589,-0.227269801620064,
0.212533521233765));
#15697=CARTESIAN_POINT('Ctrl Pts',(1.09443784939331,-0.177024326825049,
0.256354979351213));
#15698=CARTESIAN_POINT('Ctrl Pts',(1.08940878963422,-0.144299303100741,
0.276273267473431));
#15699=CARTESIAN_POINT('Ctrl Pts',(1.08431331394788,-0.0928409665394228,
0.2953917518996));
#15700=CARTESIAN_POINT('Ctrl Pts',(1.0830271513892,-0.0762225747374255,
0.300028012588062));
#15701=CARTESIAN_POINT('Ctrl Pts',(1.08212377959455,-0.0595300000000001,
0.303251606722892));
#15702=CARTESIAN_POINT('Origin',(0.,-0.05953,0.));
#15703=CARTESIAN_POINT('Origin',(0.,-0.05953,0.));
#15704=CARTESIAN_POINT('',(0.0589974094846122,-0.05953,1.07456964270265));
#15705=CARTESIAN_POINT('Origin',(0.,-0.05953,0.));
#15706=CARTESIAN_POINT('Origin',(-0.244773027351946,-0.05953,1.07242070340001));
#15707=CARTESIAN_POINT('Origin',(-0.244773027351946,0.,1.07242070340001));
#15708=CARTESIAN_POINT('',(-0.519393123750572,-0.05953,0.942555777842682));
#15709=CARTESIAN_POINT('Ctrl Pts',(-0.519393123750572,-0.05953,0.942555777842682));
#15710=CARTESIAN_POINT('Ctrl Pts',(-0.513714466572041,-0.0925528133349865,
0.945684988399766));
#15711=CARTESIAN_POINT('Ctrl Pts',(-0.503136848051455,-0.124911173756694,
0.951483858396181));
#15712=CARTESIAN_POINT('Ctrl Pts',(-0.47593627990192,-0.177924977804098,
0.965323333309091));
#15713=CARTESIAN_POINT('Ctrl Pts',(-0.460931856495794,-0.199697230012983,
0.972669835243841));
#15714=CARTESIAN_POINT('Ctrl Pts',(-0.426157505475872,-0.237895043532788,
0.988400002689705));
#15715=CARTESIAN_POINT('Ctrl Pts',(-0.406380688682952,-0.254319232363049,
0.996771768218699));
#15716=CARTESIAN_POINT('Ctrl Pts',(-0.364750145543744,-0.28018331644634,
1.01272583306292));
#15717=CARTESIAN_POINT('Ctrl Pts',(-0.340838910881557,-0.29104845371857,
1.02112815447116));
#15718=CARTESIAN_POINT('Ctrl Pts',(-0.290495481564827,-0.30527573347708,
1.036574285215));
#15719=CARTESIAN_POINT('Ctrl Pts',(-0.264056468041074,-0.308638795020976,
1.04359501395068));
#15720=CARTESIAN_POINT('Ctrl Pts',(-0.214892249704082,-0.308638795020976,
1.05481642595959));
#15721=CARTESIAN_POINT('Ctrl Pts',(-0.188025341585962,-0.30527573347708,
1.05996242598502));
#15722=CARTESIAN_POINT('Ctrl Pts',(-0.135965654106109,-0.29104845371857,
1.06788913840721));
#15723=CARTESIAN_POINT('Ctrl Pts',(-0.110776745452494,-0.28018331644634,
1.07069360430242));
#15724=CARTESIAN_POINT('Ctrl Pts',(-0.0663467128214646,-0.254319232363049,
1.07438230428002));
#15725=CARTESIAN_POINT('Ctrl Pts',(-0.0448960436540983,-0.237895043532788,
1.07542044338697));
#15726=CARTESIAN_POINT('Ctrl Pts',(-0.00674037211528124,-0.199697230012983,
1.07633607767727));
#15727=CARTESIAN_POINT('Ctrl Pts',(0.00996567398334777,-0.177924977804098,
1.07622728347683));
#15728=CARTESIAN_POINT('Ctrl Pts',(0.0404772621979741,-0.124911173756694,
1.07556023164702));
#15729=CARTESIAN_POINT('Ctrl Pts',(0.0525234025782719,-0.0925528133349865,
1.07492508698591));
#15730=CARTESIAN_POINT('Ctrl Pts',(0.0589974094846124,-0.05953,1.07456964270265));
#15731=CARTESIAN_POINT('Origin',(-0.244773027351946,-0.05953,1.07242070340001));
#15732=CARTESIAN_POINT('Origin',(0.,-0.05953,0.));
#15733=CARTESIAN_POINT('',(-0.803348093619616,-0.05953,0.716109245731214));
#15734=CARTESIAN_POINT('Origin',(0.,-0.05953,0.));
#15735=CARTESIAN_POINT('Origin',(-0.991065754692661,-0.05953,0.477272113029314));
#15736=CARTESIAN_POINT('Origin',(-0.991065754692661,0.,0.477272113029314));
#15737=CARTESIAN_POINT('',(-1.06075609691358,-0.05953,0.181596019242328));
#15738=CARTESIAN_POINT('Ctrl Pts',(-1.06075609691358,-0.05953,0.181596019242328));
#15739=CARTESIAN_POINT('Ctrl Pts',(-1.05966202740332,-0.0925528133349865,
0.187986803072856));
#15740=CARTESIAN_POINT('Ctrl Pts',(-1.05760072925372,-0.124911173756694,
0.199872254546857));
#15741=CARTESIAN_POINT('Ctrl Pts',(-1.05146158959546,-0.177924977804098,
0.22976728653846));
#15742=CARTESIAN_POINT('Ctrl Pts',(-1.04785021111757,-0.199697230012983,
0.246078686169301));
#15743=CARTESIAN_POINT('Ctrl Pts',(-1.03846709802406,-0.237895043532788,
0.283073967563097));
#15744=CARTESIAN_POINT('Ctrl Pts',(-1.03268176429485,-0.254319232363049,
0.303755815985685));
#15745=CARTESIAN_POINT('Ctrl Pts',(-1.01919893537026,-0.28018331644634,
0.346251081972725));
#15746=CARTESIAN_POINT('Ctrl Pts',(-1.01085972381132,-0.29104845371857,
0.370184399726282));
#15747=CARTESIAN_POINT('Ctrl Pts',(-0.99154738033959,-0.30527573347708,
0.419174982698463));
#15748=CARTESIAN_POINT('Ctrl Pts',(-0.980551951791748,-0.308638795020976,
0.444223188605045));
#15749=CARTESIAN_POINT('Ctrl Pts',(-0.958671816228589,-0.308638795020976,
0.489657758261848));
#15750=CARTESIAN_POINT('Ctrl Pts',(-0.945943877838127,-0.30527573347708,
0.51387163140139));
#15751=CARTESIAN_POINT('Ctrl Pts',(-0.91968254693063,-0.29104845371857,
0.559515758398093));
#15752=CARTESIAN_POINT('Ctrl Pts',(-0.906170138993533,-0.28018331644634,
0.580957796077825));
#15753=CARTESIAN_POINT('Ctrl Pts',(-0.8813524085237,-0.254319232363049,
0.617994461173994));
#15754=CARTESIAN_POINT('Ctrl Pts',(-0.868789784891799,-0.237895043532788,
0.635412538795143));
#15755=CARTESIAN_POINT('Ctrl Pts',(-0.845715984518854,-0.199697230012983,
0.66581473268113));
#15756=CARTESIAN_POINT('Ctrl Pts',(-0.835214876415962,-0.177924977804098,
0.678808213394124));
#15757=CARTESIAN_POINT('Ctrl Pts',(-0.815669690204649,-0.124911173756694,
0.702247233627224));
#15758=CARTESIAN_POINT('Ctrl Pts',(-0.807662468433796,-0.0925528133349865,
0.711269279199861));
#15759=CARTESIAN_POINT('Ctrl Pts',(-0.803348093619616,-0.05953,0.716109245731214));
#15760=CARTESIAN_POINT('Origin',(-0.991065754692661,-0.05953,0.477272113029314));
#15761=CARTESIAN_POINT('Origin',(0.,-0.05953,0.));
#15762=CARTESIAN_POINT('',(-1.076188,-0.05953,1.31795018948079E-16));
#15763=CARTESIAN_POINT('Origin',(0.,-0.05953,0.));
#15764=CARTESIAN_POINT('',(-1.06075609691358,-0.05953,-0.181596019242328));
#15765=CARTESIAN_POINT('Origin',(0.,-0.05953,0.));
#15766=CARTESIAN_POINT('Origin',(-0.991065754692661,-0.05953,-0.477272113029314));
#15767=CARTESIAN_POINT('Origin',(-0.991065754692661,0.,-0.477272113029314));
#15768=CARTESIAN_POINT('',(-0.803348093619616,-0.05953,-0.716109245731215));
#15769=CARTESIAN_POINT('Ctrl Pts',(-0.803348093619616,-0.05953,-0.716109245731215));
#15770=CARTESIAN_POINT('Ctrl Pts',(-0.807662468433795,-0.0925528133349865,
-0.711269279199862));
#15771=CARTESIAN_POINT('Ctrl Pts',(-0.815669690204649,-0.124911173756694,
-0.702247233627224));
#15772=CARTESIAN_POINT('Ctrl Pts',(-0.835214876415962,-0.177924977804098,
-0.678808213394124));
#15773=CARTESIAN_POINT('Ctrl Pts',(-0.845715984518854,-0.199697230012983,
-0.66581473268113));
#15774=CARTESIAN_POINT('Ctrl Pts',(-0.868789784891799,-0.237895043532788,
-0.635412538795143));
#15775=CARTESIAN_POINT('Ctrl Pts',(-0.8813524085237,-0.254319232363049,
-0.617994461173994));
#15776=CARTESIAN_POINT('Ctrl Pts',(-0.906170138993533,-0.28018331644634,
-0.580957796077826));
#15777=CARTESIAN_POINT('Ctrl Pts',(-0.91968254693063,-0.29104845371857,
-0.559515758398093));
#15778=CARTESIAN_POINT('Ctrl Pts',(-0.945943877838127,-0.30527573347708,
-0.51387163140139));
#15779=CARTESIAN_POINT('Ctrl Pts',(-0.958671816228589,-0.308638795020976,
-0.489657758261848));
#15780=CARTESIAN_POINT('Ctrl Pts',(-0.980551951791748,-0.308638795020976,
-0.444223188605045));
#15781=CARTESIAN_POINT('Ctrl Pts',(-0.99154738033959,-0.30527573347708,
-0.419174982698463));
#15782=CARTESIAN_POINT('Ctrl Pts',(-1.01085972381132,-0.29104845371857,
-0.370184399726282));
#15783=CARTESIAN_POINT('Ctrl Pts',(-1.01919893537026,-0.28018331644634,
-0.346251081972725));
#15784=CARTESIAN_POINT('Ctrl Pts',(-1.03268176429485,-0.254319232363049,
-0.303755815985685));
#15785=CARTESIAN_POINT('Ctrl Pts',(-1.03846709802406,-0.237895043532788,
-0.283073967563097));
#15786=CARTESIAN_POINT('Ctrl Pts',(-1.04785021111757,-0.199697230012983,
-0.246078686169302));
#15787=CARTESIAN_POINT('Ctrl Pts',(-1.05146158959546,-0.177924977804098,
-0.229767286538461));
#15788=CARTESIAN_POINT('Ctrl Pts',(-1.05760072925372,-0.124911173756694,
-0.199872254546858));
#15789=CARTESIAN_POINT('Ctrl Pts',(-1.05966202740332,-0.0925528133349864,
-0.187986803072857));
#15790=CARTESIAN_POINT('Ctrl Pts',(-1.06075609691358,-0.05953,-0.181596019242328));
#15791=CARTESIAN_POINT('Origin',(-0.991065754692661,-0.05953,-0.477272113029314));
#15792=CARTESIAN_POINT('Origin',(0.,-0.05953,0.));
#15793=CARTESIAN_POINT('',(-0.519393123750572,-0.05953,-0.942555777842682));
#15794=CARTESIAN_POINT('Origin',(0.,-0.05953,0.));
#15795=CARTESIAN_POINT('Origin',(-0.244773027351946,-0.05953,-1.07242070340001));
#15796=CARTESIAN_POINT('Origin',(-0.244773027351946,0.,-1.07242070340001));
#15797=CARTESIAN_POINT('',(0.0589974094846125,-0.05953,-1.07456964270265));
#15798=CARTESIAN_POINT('Ctrl Pts',(0.0589974094846127,-0.05953,-1.07456964270265));
#15799=CARTESIAN_POINT('Ctrl Pts',(0.0525234025782722,-0.0925528133349865,
-1.07492508698591));
#15800=CARTESIAN_POINT('Ctrl Pts',(0.0404772621979744,-0.124911173756694,
-1.07556023164702));
#15801=CARTESIAN_POINT('Ctrl Pts',(0.0099656739833481,-0.177924977804098,
-1.07622728347683));
#15802=CARTESIAN_POINT('Ctrl Pts',(-0.00674037211528096,-0.199697230012983,
-1.07633607767727));
#15803=CARTESIAN_POINT('Ctrl Pts',(-0.044896043654098,-0.237895043532788,
-1.07542044338697));
#15804=CARTESIAN_POINT('Ctrl Pts',(-0.0663467128214644,-0.254319232363049,
-1.07438230428002));
#15805=CARTESIAN_POINT('Ctrl Pts',(-0.110776745452493,-0.28018331644634,
-1.07069360430242));
#15806=CARTESIAN_POINT('Ctrl Pts',(-0.135965654106109,-0.29104845371857,
-1.06788913840721));
#15807=CARTESIAN_POINT('Ctrl Pts',(-0.188025341585962,-0.30527573347708,
-1.05996242598502));
#15808=CARTESIAN_POINT('Ctrl Pts',(-0.214892249704082,-0.308638795020976,
-1.05481642595959));
#15809=CARTESIAN_POINT('Ctrl Pts',(-0.264056468041074,-0.308638795020976,
-1.04359501395068));
#15810=CARTESIAN_POINT('Ctrl Pts',(-0.290495481564827,-0.30527573347708,
-1.036574285215));
#15811=CARTESIAN_POINT('Ctrl Pts',(-0.340838910881557,-0.291048453718569,
-1.02112815447116));
#15812=CARTESIAN_POINT('Ctrl Pts',(-0.364750145543744,-0.28018331644634,
-1.01272583306292));
#15813=CARTESIAN_POINT('Ctrl Pts',(-0.406380688682952,-0.254319232363049,
-0.996771768218699));
#15814=CARTESIAN_POINT('Ctrl Pts',(-0.426157505475872,-0.237895043532788,
-0.988400002689705));
#15815=CARTESIAN_POINT('Ctrl Pts',(-0.460931856495794,-0.199697230012983,
-0.972669835243841));
#15816=CARTESIAN_POINT('Ctrl Pts',(-0.475936279901919,-0.177924977804098,
-0.965323333309091));
#15817=CARTESIAN_POINT('Ctrl Pts',(-0.503136848051454,-0.124911173756694,
-0.951483858396181));
#15818=CARTESIAN_POINT('Ctrl Pts',(-0.513714466572041,-0.0925528133349865,
-0.945684988399766));
#15819=CARTESIAN_POINT('Ctrl Pts',(-0.519393123750572,-0.05953,-0.942555777842682));
#15820=CARTESIAN_POINT('Origin',(-0.244773027351946,-0.05953,-1.07242070340001));
#15821=CARTESIAN_POINT('Origin',(0.,-0.05953,0.));
#15822=CARTESIAN_POINT('',(0.413083465285518,-0.05953,-0.993751811093549));
#15823=CARTESIAN_POINT('Origin',(0.,-0.05953,0.));
#15824=CARTESIAN_POINT('Origin',(0.685838782044607,-0.05953,-0.860014630714833));
#15825=CARTESIAN_POINT('Origin',(0.685838782044607,0.,-0.860014630714833));
#15826=CARTESIAN_POINT('',(0.876916659919095,-0.05953,-0.623857181492959));
#15827=CARTESIAN_POINT('Ctrl Pts',(0.876916659919095,-0.05953,-0.623857181492958));
#15828=CARTESIAN_POINT('Ctrl Pts',(0.873158080166742,-0.0925528133349865,
-0.62914037979579));
#15829=CARTESIAN_POINT('Ctrl Pts',(0.866144010579847,-0.124911173756694,
-0.638954437806245));
#15830=CARTESIAN_POINT('Ctrl Pts',(0.847641868610495,-0.177924977804098,
-0.663225258065736));
#15831=CARTESIAN_POINT('Ctrl Pts',(0.837310877969633,-0.199697230012983,
-0.676354402927683));
#15832=CARTESIAN_POINT('Ctrl Pts',(0.81280533416753,-0.237895043532788,
-0.705614819529209));
#15833=CARTESIAN_POINT('Ctrl Pts',(0.798619410861634,-0.254319232363049,
-0.721738358858166));
#15834=CARTESIAN_POINT('Ctrl Pts',(0.768033796848072,-0.28018331644634,
-0.754175290318038));
#15835=CARTESIAN_POINT('Ctrl Pts',(0.750136149454208,-0.29104845371857,
-0.772120216227122));
#15836=CARTESIAN_POINT('Ctrl Pts',(0.711480111898423,-0.30527573347708,
-0.807879894508811));
#15837=CARTESIAN_POINT('Ctrl Pts',(0.690705563850638,-0.308638795020976,
-0.825676810575913));
#15838=CARTESIAN_POINT('Ctrl Pts',(0.651278921914856,-0.308638795020976,
-0.857118508332695));
#15839=CARTESIAN_POINT('Ctrl Pts',(0.629305439856167,-0.30527573347708,
-0.873412008702649));
#15840=CARTESIAN_POINT('Ctrl Pts',(0.585840553788742,-0.29104845371857,
-0.903141581680914));
#15841=CARTESIAN_POINT('Ctrl Pts',(0.564362943424239,-0.28018331644634,
-0.916597376014514));
#15842=CARTESIAN_POINT('Ctrl Pts',(0.525933334162556,-0.254319232363049,
-0.939198248544427));
#15843=CARTESIAN_POINT('Ctrl Pts',(0.507057380724533,-0.237895043532788,
-0.949440676105255));
#15844=CARTESIAN_POINT('Ctrl Pts',(0.473077587363686,-0.199697230012983,
-0.966820759530997));
#15845=CARTESIAN_POINT('Ctrl Pts',(0.457978755888596,-0.177924977804098,
-0.973971221090534));
#15846=CARTESIAN_POINT('Ctrl Pts',(0.430199341854858,-0.124911173756694,
-0.986608710139579));
#15847=CARTESIAN_POINT('Ctrl Pts',(0.419070565453384,-0.0925528133349865,
-0.991263089003441));
#15848=CARTESIAN_POINT('Ctrl Pts',(0.413083465285518,-0.05953,-0.993751811093549));
#15849=CARTESIAN_POINT('Origin',(0.685838782044607,-0.05953,-0.860014630714833));
#15850=CARTESIAN_POINT('Origin',(0.,-0.208355,0.));
#15851=CARTESIAN_POINT('',(-1.076188,-0.35718,1.31795018948079E-16));
#15852=CARTESIAN_POINT('Origin',(0.,-0.35718,0.));
#15853=CARTESIAN_POINT('',(-1.076188,-0.208355,1.31795018948079E-16));
#15854=CARTESIAN_POINT('',(1.03449977959455,-0.05953,0.296632461748266));
#15855=CARTESIAN_POINT('Origin',(0.,-0.05953,0.));
#15856=CARTESIAN_POINT('',(1.03449977959455,-0.05953,-0.296632461748266));
#15857=CARTESIAN_POINT('Ctrl Pts',(1.03449977959455,-0.05953,0.296632461748267));
#15858=CARTESIAN_POINT('Ctrl Pts',(1.03628691421076,-0.0925528133349865,
0.290399865505497));
#15859=CARTESIAN_POINT('Ctrl Pts',(1.03958665287714,-0.124911173756694,
0.278797079997872));
#15860=CARTESIAN_POINT('Ctrl Pts',(1.0470264474309,-0.177924977804098,0.249198913998601));
#15861=CARTESIAN_POINT('Ctrl Pts',(1.05084995891418,-0.199697230012983,
0.232935932341942));
#15862=CARTESIAN_POINT('Ctrl Pts',(1.05844771715377,-0.237895043532788,
0.195533155353269));
#15863=CARTESIAN_POINT('Ctrl Pts',(1.06220882929878,-0.254319232363049,
0.17438929156337));
#15864=CARTESIAN_POINT('Ctrl Pts',(1.06849922508772,-0.28018331644634,0.130252399648131));
#15865=CARTESIAN_POINT('Ctrl Pts',(1.07137013248666,-0.29104845371857,0.105070977154072));
#15866=CARTESIAN_POINT('Ctrl Pts',(1.07522652957392,-0.30527573347708,0.0525526752791107));
#15867=CARTESIAN_POINT('Ctrl Pts',(1.076188,-0.308638795020976,0.025214283908933));
#15868=CARTESIAN_POINT('Ctrl Pts',(1.076188,-0.308638795020976,-0.025214283908933));
#15869=CARTESIAN_POINT('Ctrl Pts',(1.07522652957392,-0.30527573347708,-0.0525526752791107));
#15870=CARTESIAN_POINT('Ctrl Pts',(1.07137013248666,-0.29104845371857,-0.105070977154072));
#15871=CARTESIAN_POINT('Ctrl Pts',(1.06849922508772,-0.28018331644634,-0.130252399648131));
#15872=CARTESIAN_POINT('Ctrl Pts',(1.06220882929878,-0.254319232363049,
-0.17438929156337));
#15873=CARTESIAN_POINT('Ctrl Pts',(1.05844771715377,-0.237895043532788,
-0.195533155353269));
#15874=CARTESIAN_POINT('Ctrl Pts',(1.05084995891418,-0.199697230012983,
-0.232935932341942));
#15875=CARTESIAN_POINT('Ctrl Pts',(1.0470264474309,-0.177924977804098,-0.249198913998601));
#15876=CARTESIAN_POINT('Ctrl Pts',(1.03958665287714,-0.124911173756694,
-0.278797079997872));
#15877=CARTESIAN_POINT('Ctrl Pts',(1.03628691421076,-0.0925528133349865,
-0.290399865505497));
#15878=CARTESIAN_POINT('Ctrl Pts',(1.03449977959455,-0.05953,-0.296632461748267));
#15879=CARTESIAN_POINT('Origin',(0.,-0.05953,0.));
#15880=CARTESIAN_POINT('Origin',(0.,-0.05953,0.));
#15881=CARTESIAN_POINT('Origin',(1.1,-0.05953,0.));
#15882=CARTESIAN_POINT('Origin',(1.1,0.,0.));
#15883=CARTESIAN_POINT('Origin',(1.1,-0.05953,0.));
#15884=CARTESIAN_POINT('Origin',(0.,-0.35718,0.));
#15885=CARTESIAN_POINT('Origin',(0.,-0.05953,0.));
#16971=UNCERTAINTY_MEASURE_WITH_UNIT(LENGTH_MEASURE(0.001),#17047,
'DISTANCE_ACCURACY_VALUE',
'Maximum model space distance between geometric entities at asserted c
onnectivities');
#16993=UNCERTAINTY_MEASURE_WITH_UNIT(LENGTH_MEASURE(0.001),#17047,
'DISTANCE_ACCURACY_VALUE',
'Maximum model space distance between geometric entities at asserted c
onnectivities');
#17024=(
GEOMETRIC_REPRESENTATION_CONTEXT(3)
GLOBAL_UNCERTAINTY_ASSIGNED_CONTEXT((#16971))
GLOBAL_UNIT_ASSIGNED_CONTEXT((#17047,#17049,#17050))
REPRESENTATION_CONTEXT('','3D')
);
#17046=(
GEOMETRIC_REPRESENTATION_CONTEXT(3)
GLOBAL_UNCERTAINTY_ASSIGNED_CONTEXT((#16993))
GLOBAL_UNIT_ASSIGNED_CONTEXT((#17047,#17049,#17050))
REPRESENTATION_CONTEXT('','3D')
);
#17047=(
LENGTH_UNIT()
NAMED_UNIT(*)
SI_UNIT(.CENTI.,.METRE.)
);
#17049=(
NAMED_UNIT(*)
PLANE_ANGLE_UNIT()
SI_UNIT($,.RADIAN.)
);
#17050=(
NAMED_UNIT(*)
SI_UNIT($,.STERADIAN.)
SOLID_ANGLE_UNIT()
);
#17081=SHAPE_DEFINITION_REPRESENTATION(#17133,#17288);
#17133=PRODUCT_DEFINITION_SHAPE('',$,#17341);
#17288=SHAPE_REPRESENTATION('',(#9317),#17024);
#17310=PRODUCT_DEFINITION_CONTEXT('part definition',#17468,'design');
#17341=PRODUCT_DEFINITION('Cage','Cage',#17393,#17310);
#17393=PRODUCT_DEFINITION_FORMATION('',$,#17500);
#17468=APPLICATION_CONTEXT(
'Core Data for Automotive Mechanical Design Process');
#17469=PRODUCT_CONTEXT('part definition',#17468,'mechanical');
#17500=PRODUCT('Cage','Cage','Cage',(#17469));
#17585=COLOUR_RGB('Grey',0.48,0.52,0.57);
#17586=FILL_AREA_STYLE_COLOUR('',#17585);
#17587=FILL_AREA_STYLE('',(#17586));
#17588=SURFACE_STYLE_FILL_AREA(#17587);
#17589=SURFACE_SIDE_STYLE('',(#17588));
#17590=SURFACE_STYLE_USAGE(.BOTH.,#17589);
#17591=PRESENTATION_STYLE_ASSIGNMENT((#17590));
ENDSEC;
END-ISO-10303-21;
